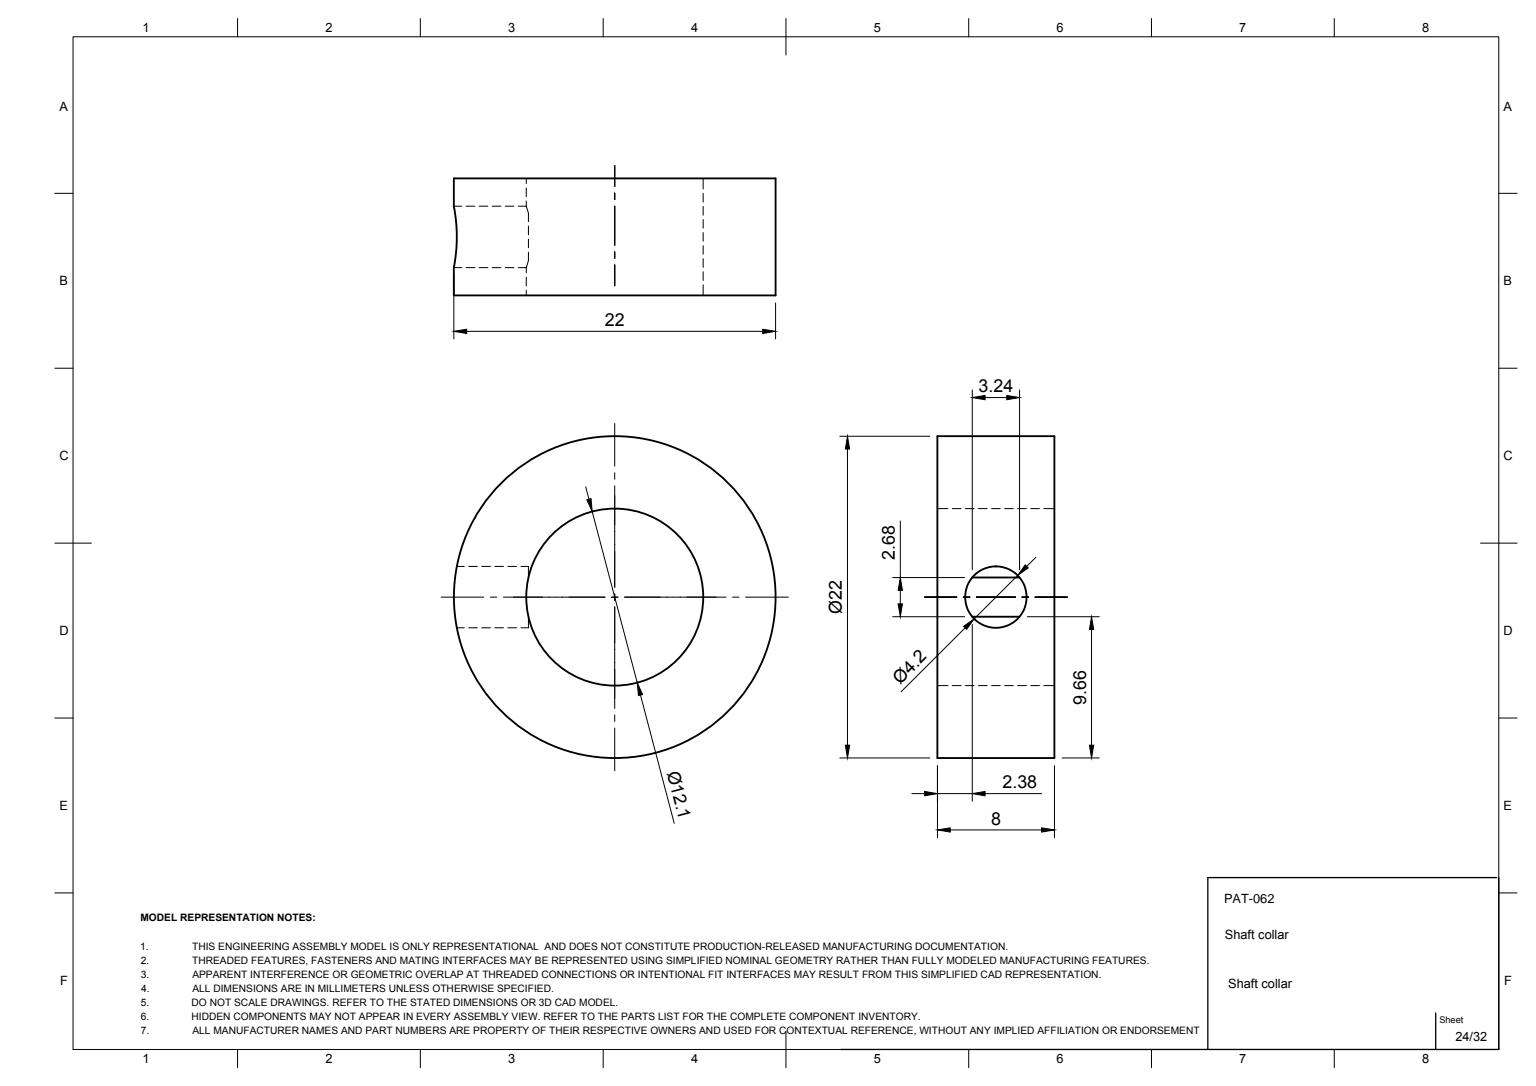
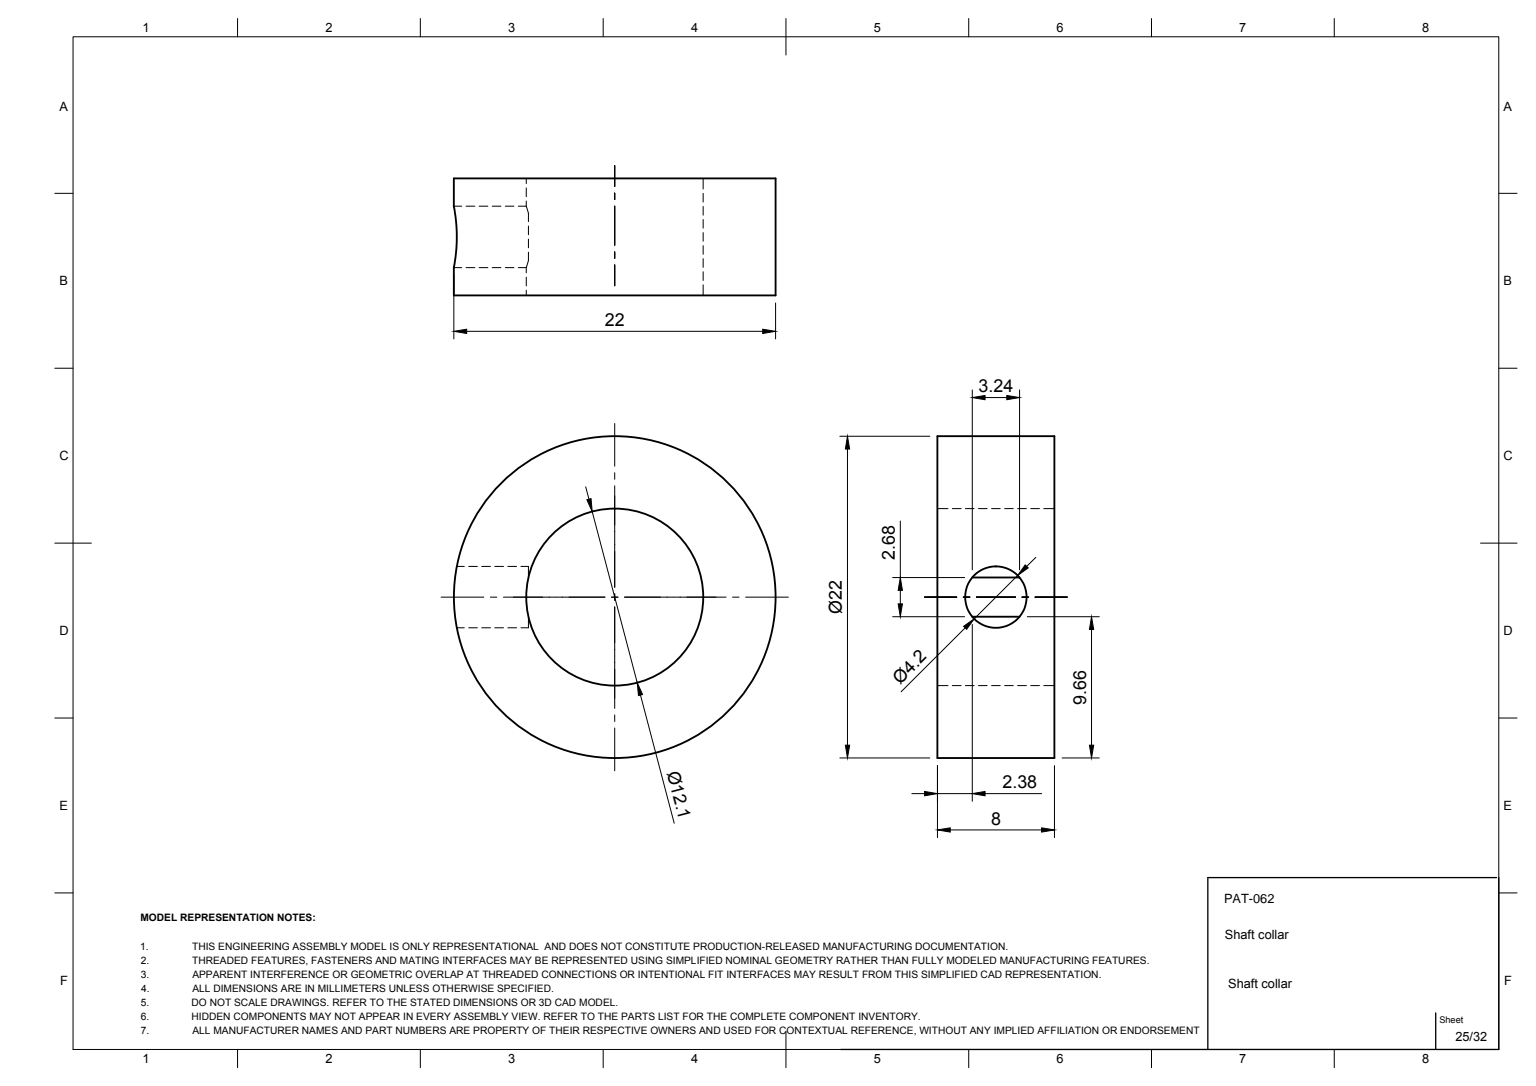
ISO-10303-21;
HEADER;
/* Generated by software containing ST-Developer
 * from STEP Tools, Inc. (www.steptools.com) 
 */

FILE_DESCRIPTION(
/* description */ ('Jaw-coupled motor to shaft test stand'),
/* implementation_level */ '2;1');

FILE_NAME(
/* name */ 'Shaft collar.step',
/* time_stamp */ '2026-10-27T10:46:06-07:00',
/* author */ (''),
/* organization */ (''),
/* preprocessor_version */ 'ST-DEVELOPER v20.2',
/* originating_system */ 'Autodesk Translation Framework v15.17.0.0',
/* authorisation */ '');

FILE_SCHEMA (('AUTOMOTIVE_DESIGN { 1 0 10303 214 3 1 1 }'));
ENDSEC;

DATA;
#10=MECHANICAL_DESIGN_GEOMETRIC_PRESENTATION_REPRESENTATION('',(#363),#19361);
#259=B_SPLINE_CURVE_WITH_KNOTS('',3,(#17076,#17077,#17078,#17079,#17080,
#17081,#17082,#17083,#17084,#17085),.UNSPECIFIED.,.F.,.F.,(4,2,2,2,4),(0.818088904349167,
0.878131747417164,0.957937926194035,1.03774410497091,1.0977869480389),
 .UNSPECIFIED.);
#260=B_SPLINE_CURVE_WITH_KNOTS('',3,(#17091,#17092,#17093,#17094,#17095,
#17096,#17097,#17098,#17099,#17100,#17101,#17102,#17103,#17104,#17105,#17106,
#17107,#17108),.UNSPECIFIED.,.F.,.F.,(4,2,2,2,2,2,2,2,4),(0.,0.0793157643915217,
0.158631528783043,0.237943615933649,0.317255703084255,0.396567790234861,
0.475879877385467,0.555195641776989,0.63451140616851),.UNSPECIFIED.);
#261=B_SPLINE_CURVE_WITH_KNOTS('',3,(#17109,#17110,#17111,#17112,#17113,
#17114,#17115,#17116,#17117,#17118,#17119,#17120,#17121,#17122,#17123,#17124,
#17125,#17126),.UNSPECIFIED.,.F.,.F.,(4,2,2,2,2,2,2,2,4),(0.63451140616851,
0.713827170560032,0.793142934951554,0.87245502210216,0.951767109252766,
1.03107919640337,1.11039128355398,1.1897070479455,1.26902281233702),
 .UNSPECIFIED.);
#262=B_SPLINE_CURVE_WITH_KNOTS('',3,(#17129,#17130,#17131,#17132,#17133,
#17134,#17135,#17136,#17137,#17138),.UNSPECIFIED.,.F.,.F.,(4,2,2,2,4),(0.179463620219811,
0.239506463287807,0.319312642064678,0.399118820841549,0.459161663909546),
 .UNSPECIFIED.);
#298=SHAPE_REPRESENTATION_RELATIONSHIP('SRR','None',#19514,#330);
#330=ADVANCED_BREP_SHAPE_REPRESENTATION('',(#394),#19350);
#363=STYLED_ITEM('',(#19746),#394);
#394=MANIFOLD_SOLID_BREP('Body1',#11009);
#495=FACE_BOUND('',#1973,.T.);
#496=FACE_BOUND('',#1975,.T.);
#497=FACE_BOUND('',#1977,.T.);
#498=FACE_BOUND('',#1979,.T.);
#675=PLANE('',#11808);
#676=PLANE('',#11813);
#677=PLANE('',#11820);
#678=PLANE('',#11821);
#1257=FACE_OUTER_BOUND('',#1969,.T.);
#1258=FACE_OUTER_BOUND('',#1970,.T.);
#1259=FACE_OUTER_BOUND('',#1971,.T.);
#1260=FACE_OUTER_BOUND('',#1972,.T.);
#1261=FACE_OUTER_BOUND('',#1974,.T.);
#1262=FACE_OUTER_BOUND('',#1976,.T.);
#1263=FACE_OUTER_BOUND('',#1978,.T.);
#1969=EDGE_LOOP('',(#8348,#8349));
#1970=EDGE_LOOP('',(#8350,#8351,#8352,#8353,#8354,#8355,#8356,#8357,#8358));
#1971=EDGE_LOOP('',(#8359,#8360,#8361));
#1972=EDGE_LOOP('',(#8362,#8363,#8364,#8365));
#1973=EDGE_LOOP('',(#8366,#8367,#8368,#8369));
#1974=EDGE_LOOP('',(#8370,#8371,#8372,#8373));
#1975=EDGE_LOOP('',(#8374,#8375));
#1976=EDGE_LOOP('',(#8376));
#1977=EDGE_LOOP('',(#8377));
#1978=EDGE_LOOP('',(#8378));
#1979=EDGE_LOOP('',(#8379));
#2698=LINE('',#17072,#3851);
#2699=LINE('',#17089,#3852);
#2700=LINE('',#17140,#3853);
#2701=LINE('',#17145,#3854);
#2702=LINE('',#17151,#3855);
#3851=VECTOR('',#13535,1.);
#3852=VECTOR('',#13542,0.21);
#3853=VECTOR('',#13547,1.);
#3854=VECTOR('',#13552,0.605);
#3855=VECTOR('',#13559,1.1);
#4827=CIRCLE('',#11809,0.21);
#4828=CIRCLE('',#11811,0.21);
#4829=CIRCLE('',#11812,0.21);
#4830=CIRCLE('',#11815,0.605);
#4831=CIRCLE('',#11816,0.605);
#4832=CIRCLE('',#11818,1.1);
#4833=CIRCLE('',#11819,1.1);
#5283=VERTEX_POINT('',#17070);
#5284=VERTEX_POINT('',#17071);
#5285=VERTEX_POINT('',#17075);
#5286=VERTEX_POINT('',#17086);
#5287=VERTEX_POINT('',#17088);
#5288=VERTEX_POINT('',#17090);
#5289=VERTEX_POINT('',#17127);
#5290=VERTEX_POINT('',#17142);
#5291=VERTEX_POINT('',#17144);
#5292=VERTEX_POINT('',#17148);
#5293=VERTEX_POINT('',#17150);
#6385=EDGE_CURVE('',#5283,#5284,#2698,.T.);
#6386=EDGE_CURVE('',#5283,#5284,#4827,.T.);
#6387=EDGE_CURVE('',#5285,#5283,#259,.T.);
#6388=EDGE_CURVE('',#5286,#5285,#4828,.T.);
#6389=EDGE_CURVE('',#5286,#5287,#2699,.T.);
#6390=EDGE_CURVE('',#5288,#5287,#260,.T.);
#6391=EDGE_CURVE('',#5287,#5288,#261,.T.);
#6392=EDGE_CURVE('',#5289,#5286,#4829,.T.);
#6393=EDGE_CURVE('',#5284,#5289,#262,.T.);
#6394=EDGE_CURVE('',#5289,#5285,#2700,.T.);
#6395=EDGE_CURVE('',#5290,#5290,#4830,.T.);
#6396=EDGE_CURVE('',#5290,#5291,#2701,.T.);
#6397=EDGE_CURVE('',#5291,#5291,#4831,.T.);
#6398=EDGE_CURVE('',#5292,#5292,#4832,.T.);
#6399=EDGE_CURVE('',#5292,#5293,#2702,.T.);
#6400=EDGE_CURVE('',#5293,#5293,#4833,.T.);
#8348=ORIENTED_EDGE('',*,*,#6385,.F.);
#8349=ORIENTED_EDGE('',*,*,#6386,.T.);
#8350=ORIENTED_EDGE('',*,*,#6387,.F.);
#8351=ORIENTED_EDGE('',*,*,#6388,.F.);
#8352=ORIENTED_EDGE('',*,*,#6389,.T.);
#8353=ORIENTED_EDGE('',*,*,#6390,.F.);
#8354=ORIENTED_EDGE('',*,*,#6391,.F.);
#8355=ORIENTED_EDGE('',*,*,#6389,.F.);
#8356=ORIENTED_EDGE('',*,*,#6392,.F.);
#8357=ORIENTED_EDGE('',*,*,#6393,.F.);
#8358=ORIENTED_EDGE('',*,*,#6386,.F.);
#8359=ORIENTED_EDGE('',*,*,#6394,.F.);
#8360=ORIENTED_EDGE('',*,*,#6392,.T.);
#8361=ORIENTED_EDGE('',*,*,#6388,.T.);
#8362=ORIENTED_EDGE('',*,*,#6395,.F.);
#8363=ORIENTED_EDGE('',*,*,#6396,.T.);
#8364=ORIENTED_EDGE('',*,*,#6397,.T.);
#8365=ORIENTED_EDGE('',*,*,#6396,.F.);
#8366=ORIENTED_EDGE('',*,*,#6393,.T.);
#8367=ORIENTED_EDGE('',*,*,#6394,.T.);
#8368=ORIENTED_EDGE('',*,*,#6387,.T.);
#8369=ORIENTED_EDGE('',*,*,#6385,.T.);
#8370=ORIENTED_EDGE('',*,*,#6398,.F.);
#8371=ORIENTED_EDGE('',*,*,#6399,.T.);
#8372=ORIENTED_EDGE('',*,*,#6400,.T.);
#8373=ORIENTED_EDGE('',*,*,#6399,.F.);
#8374=ORIENTED_EDGE('',*,*,#6390,.T.);
#8375=ORIENTED_EDGE('',*,*,#6391,.T.);
#8376=ORIENTED_EDGE('',*,*,#6398,.T.);
#8377=ORIENTED_EDGE('',*,*,#6395,.T.);
#8378=ORIENTED_EDGE('',*,*,#6400,.F.);
#8379=ORIENTED_EDGE('',*,*,#6397,.F.);
#10338=CYLINDRICAL_SURFACE('',#11810,0.21);
#10339=CYLINDRICAL_SURFACE('',#11814,0.605);
#10340=CYLINDRICAL_SURFACE('',#11817,1.1);
#10599=ADVANCED_FACE('',(#1257),#675,.T.);
#10600=ADVANCED_FACE('',(#1258),#10338,.F.);
#10601=ADVANCED_FACE('',(#1259),#676,.T.);
#10602=ADVANCED_FACE('',(#1260,#495),#10339,.F.);
#10603=ADVANCED_FACE('',(#1261,#496),#10340,.T.);
#10604=ADVANCED_FACE('',(#1262,#497),#677,.T.);
#10605=ADVANCED_FACE('',(#1263,#498),#678,.F.);
#11009=CLOSED_SHELL('',(#10599,#10600,#10601,#10602,#10603,#10604,#10605));
#11807=AXIS2_PLACEMENT_3D('',#17068,#13531,#13532);
#11808=AXIS2_PLACEMENT_3D('',#17069,#13533,#13534);
#11809=AXIS2_PLACEMENT_3D('',#17073,#13536,#13537);
#11810=AXIS2_PLACEMENT_3D('',#17074,#13538,#13539);
#11811=AXIS2_PLACEMENT_3D('',#17087,#13540,#13541);
#11812=AXIS2_PLACEMENT_3D('',#17128,#13543,#13544);
#11813=AXIS2_PLACEMENT_3D('',#17139,#13545,#13546);
#11814=AXIS2_PLACEMENT_3D('',#17141,#13548,#13549);
#11815=AXIS2_PLACEMENT_3D('',#17143,#13550,#13551);
#11816=AXIS2_PLACEMENT_3D('',#17146,#13553,#13554);
#11817=AXIS2_PLACEMENT_3D('',#17147,#13555,#13556);
#11818=AXIS2_PLACEMENT_3D('',#17149,#13557,#13558);
#11819=AXIS2_PLACEMENT_3D('',#17152,#13560,#13561);
#11820=AXIS2_PLACEMENT_3D('',#17153,#13562,#13563);
#11821=AXIS2_PLACEMENT_3D('',#17154,#13564,#13565);
#13531=DIRECTION('axis',(0.,0.,1.));
#13532=DIRECTION('refdir',(1.,0.,0.));
#13533=DIRECTION('center_axis',(0.,0.,1.));
#13534=DIRECTION('ref_axis',(1.,0.,0.));
#13535=DIRECTION('',(0.,1.,0.));
#13536=DIRECTION('center_axis',(0.,0.,1.));
#13537=DIRECTION('ref_axis',(1.,0.,0.));
#13538=DIRECTION('center_axis',(0.,0.,1.));
#13539=DIRECTION('ref_axis',(1.,0.,0.));
#13540=DIRECTION('center_axis',(0.,0.,1.));
#13541=DIRECTION('ref_axis',(1.,0.,0.));
#13542=DIRECTION('',(0.,0.,1.));
#13543=DIRECTION('center_axis',(0.,0.,1.));
#13544=DIRECTION('ref_axis',(1.,0.,0.));
#13545=DIRECTION('center_axis',(0.,0.,1.));
#13546=DIRECTION('ref_axis',(1.,0.,0.));
#13547=DIRECTION('',(0.,-1.,0.));
#13548=DIRECTION('center_axis',(0.,1.,0.));
#13549=DIRECTION('ref_axis',(1.,0.,0.));
#13550=DIRECTION('center_axis',(0.,-1.,0.));
#13551=DIRECTION('ref_axis',(1.,0.,0.));
#13552=DIRECTION('',(0.,-1.,0.));
#13553=DIRECTION('center_axis',(0.,-1.,0.));
#13554=DIRECTION('ref_axis',(1.,0.,0.));
#13555=DIRECTION('center_axis',(0.,1.,0.));
#13556=DIRECTION('ref_axis',(1.,0.,0.));
#13557=DIRECTION('center_axis',(0.,1.,0.));
#13558=DIRECTION('ref_axis',(1.,0.,0.));
#13559=DIRECTION('',(0.,-1.,0.));
#13560=DIRECTION('center_axis',(0.,1.,0.));
#13561=DIRECTION('ref_axis',(1.,0.,0.));
#13562=DIRECTION('center_axis',(0.,1.,0.));
#13563=DIRECTION('ref_axis',(1.,0.,0.));
#13564=DIRECTION('center_axis',(0.,1.,0.));
#13565=DIRECTION('ref_axis',(1.,0.,0.));
#17068=CARTESIAN_POINT('',(0.,0.,0.));
#17069=CARTESIAN_POINT('Origin',(0.,0.75,4.81));
#17070=CARTESIAN_POINT('',(0.133884278389959,0.588213103126366,4.81));
#17071=CARTESIAN_POINT('',(0.133884278389959,0.911786896873634,4.81));
#17072=CARTESIAN_POINT('',(0.133884278389959,0.35,4.81));
#17073=CARTESIAN_POINT('Origin',(0.,0.75,4.81));
#17074=CARTESIAN_POINT('Origin',(0.,0.75,4.81));
#17075=CARTESIAN_POINT('',(-0.133884278389959,0.588213103126366,4.81));
#17076=CARTESIAN_POINT('Ctrl Pts',(-0.133884278389959,0.588213103126366,
4.81));
#17077=CARTESIAN_POINT('Ctrl Pts',(-0.118254395260805,0.575278831782373,
4.81354677224418));
#17078=CARTESIAN_POINT('Ctrl Pts',(-0.1001097876823,0.564200683412563,4.81698224789957));
#17079=CARTESIAN_POINT('Ctrl Pts',(-0.0548298721325192,0.545361438945571,
4.8230741628997));
#17080=CARTESIAN_POINT('Ctrl Pts',(-0.0266020595922903,0.54,4.825));
#17081=CARTESIAN_POINT('Ctrl Pts',(0.0266020595922903,0.54,4.825));
#17082=CARTESIAN_POINT('Ctrl Pts',(0.0548298721325192,0.545361438945571,
4.8230741628997));
#17083=CARTESIAN_POINT('Ctrl Pts',(0.1001097876823,0.564200683412563,4.81698224789957));
#17084=CARTESIAN_POINT('Ctrl Pts',(0.118254395260805,0.575278831782372,
4.81354677224418));
#17085=CARTESIAN_POINT('Ctrl Pts',(0.133884278389959,0.588213103126366,
4.81));
#17086=CARTESIAN_POINT('',(-0.21,0.75,4.81));
#17087=CARTESIAN_POINT('Origin',(0.,0.75,4.81));
#17088=CARTESIAN_POINT('',(-0.21,0.75,5.29976849370594));
#17089=CARTESIAN_POINT('',(-0.21,0.75,4.81));
#17090=CARTESIAN_POINT('',(0.21,0.75,5.29976849370594));
#17091=CARTESIAN_POINT('Ctrl Pts',(0.21,0.75,5.29976849370594));
#17092=CARTESIAN_POINT('Ctrl Pts',(0.21,0.723561411869493,5.29976849370594));
#17093=CARTESIAN_POINT('Ctrl Pts',(0.204702922670976,0.695406218745069,
5.30084015664674));
#17094=CARTESIAN_POINT('Ctrl Pts',(0.183251796806354,0.643686554458656,
5.30468313707126));
#17095=CARTESIAN_POINT('Ctrl Pts',(0.167101177357214,0.620116329258865,
5.30739593054622));
#17096=CARTESIAN_POINT('Ctrl Pts',(0.129884533480965,0.582899685382615,
5.31246633289124));
#17097=CARTESIAN_POINT('Ctrl Pts',(0.106313940757289,0.566748389836589,
5.31515738895358));
#17098=CARTESIAN_POINT('Ctrl Pts',(0.0545930033295205,0.545296773430262,
5.31895039220591));
#17099=CARTESIAN_POINT('Ctrl Pts',(0.0264373623835353,0.54,5.32));
#17100=CARTESIAN_POINT('Ctrl Pts',(-0.0264373623835353,0.54,5.32));
#17101=CARTESIAN_POINT('Ctrl Pts',(-0.0545930033295205,0.545296773430262,
5.31895039220591));
#17102=CARTESIAN_POINT('Ctrl Pts',(-0.106313940757289,0.566748389836589,
5.31515738895358));
#17103=CARTESIAN_POINT('Ctrl Pts',(-0.129884533480965,0.582899685382615,
5.31246633289124));
#17104=CARTESIAN_POINT('Ctrl Pts',(-0.167101177357214,0.620116329258865,
5.30739593054622));
#17105=CARTESIAN_POINT('Ctrl Pts',(-0.183251796806354,0.643686554458656,
5.30468313707126));
#17106=CARTESIAN_POINT('Ctrl Pts',(-0.204702922670976,0.695406218745069,
5.30084015664674));
#17107=CARTESIAN_POINT('Ctrl Pts',(-0.21,0.723561411869493,5.29976849370594));
#17108=CARTESIAN_POINT('Ctrl Pts',(-0.21,0.75,5.29976849370594));
#17109=CARTESIAN_POINT('Ctrl Pts',(-0.21,0.75,5.29976849370594));
#17110=CARTESIAN_POINT('Ctrl Pts',(-0.21,0.776438588130507,5.29976849370594));
#17111=CARTESIAN_POINT('Ctrl Pts',(-0.204702922670976,0.804593781254931,
5.30084015664674));
#17112=CARTESIAN_POINT('Ctrl Pts',(-0.183251796806354,0.856313445541343,
5.30468313707126));
#17113=CARTESIAN_POINT('Ctrl Pts',(-0.167101177357215,0.879883670741135,
5.30739593054622));
#17114=CARTESIAN_POINT('Ctrl Pts',(-0.129884533480965,0.917100314617385,
5.31246633289124));
#17115=CARTESIAN_POINT('Ctrl Pts',(-0.106313940757289,0.933251610163411,
5.31515738895358));
#17116=CARTESIAN_POINT('Ctrl Pts',(-0.0545930033295205,0.954703226569738,
5.31895039220591));
#17117=CARTESIAN_POINT('Ctrl Pts',(-0.0264373623835353,0.96,5.32));
#17118=CARTESIAN_POINT('Ctrl Pts',(0.0264373623835353,0.96,5.32));
#17119=CARTESIAN_POINT('Ctrl Pts',(0.0545930033295204,0.954703226569738,
5.31895039220591));
#17120=CARTESIAN_POINT('Ctrl Pts',(0.106313940757288,0.933251610163411,
5.31515738895358));
#17121=CARTESIAN_POINT('Ctrl Pts',(0.129884533480965,0.917100314617385,
5.31246633289124));
#17122=CARTESIAN_POINT('Ctrl Pts',(0.167101177357214,0.879883670741136,
5.30739593054622));
#17123=CARTESIAN_POINT('Ctrl Pts',(0.183251796806354,0.856313445541344,
5.30468313707126));
#17124=CARTESIAN_POINT('Ctrl Pts',(0.204702922670976,0.804593781254931,
5.30084015664674));
#17125=CARTESIAN_POINT('Ctrl Pts',(0.21,0.776438588130507,5.29976849370594));
#17126=CARTESIAN_POINT('Ctrl Pts',(0.21,0.75,5.29976849370594));
#17127=CARTESIAN_POINT('',(-0.133884278389959,0.911786896873634,4.81));
#17128=CARTESIAN_POINT('Origin',(0.,0.75,4.81));
#17129=CARTESIAN_POINT('Ctrl Pts',(0.133884278389959,0.911786896873634,
4.81));
#17130=CARTESIAN_POINT('Ctrl Pts',(0.118254395260805,0.924721168217627,
4.81354677224418));
#17131=CARTESIAN_POINT('Ctrl Pts',(0.1001097876823,0.935799316587437,4.81698224789957));
#17132=CARTESIAN_POINT('Ctrl Pts',(0.0548298721325192,0.954638561054429,
4.8230741628997));
#17133=CARTESIAN_POINT('Ctrl Pts',(0.0266020595922903,0.96,4.825));
#17134=CARTESIAN_POINT('Ctrl Pts',(-0.0266020595922903,0.96,4.825));
#17135=CARTESIAN_POINT('Ctrl Pts',(-0.0548298721325192,0.954638561054429,
4.8230741628997));
#17136=CARTESIAN_POINT('Ctrl Pts',(-0.1001097876823,0.935799316587437,4.81698224789957));
#17137=CARTESIAN_POINT('Ctrl Pts',(-0.118254395260804,0.924721168217628,
4.81354677224418));
#17138=CARTESIAN_POINT('Ctrl Pts',(-0.133884278389959,0.911786896873634,
4.81));
#17139=CARTESIAN_POINT('Origin',(0.,0.75,4.81));
#17140=CARTESIAN_POINT('',(-0.133884278389959,0.35,4.81));
#17141=CARTESIAN_POINT('Origin',(0.,0.35,4.22));
#17142=CARTESIAN_POINT('',(-0.605,1.15,4.22));
#17143=CARTESIAN_POINT('Origin',(0.,1.15,4.22));
#17144=CARTESIAN_POINT('',(-0.605,0.35,4.22));
#17145=CARTESIAN_POINT('',(-0.605,0.35,4.22));
#17146=CARTESIAN_POINT('Origin',(0.,0.35,4.22));
#17147=CARTESIAN_POINT('Origin',(0.,0.35,4.22));
#17148=CARTESIAN_POINT('',(-1.1,1.15,4.22));
#17149=CARTESIAN_POINT('Origin',(0.,1.15,4.22));
#17150=CARTESIAN_POINT('',(-1.1,0.35,4.22));
#17151=CARTESIAN_POINT('',(-1.1,0.35,4.22));
#17152=CARTESIAN_POINT('Origin',(0.,0.35,4.22));
#17153=CARTESIAN_POINT('Origin',(0.,1.15,4.22));
#17154=CARTESIAN_POINT('Origin',(0.,0.35,4.22));
#19312=UNCERTAINTY_MEASURE_WITH_UNIT(LENGTH_MEASURE(0.001),#19362,
'DISTANCE_ACCURACY_VALUE',
'Maximum model space distance between geometric entities at asserted c
onnectivities');
#19323=UNCERTAINTY_MEASURE_WITH_UNIT(LENGTH_MEASURE(0.001),#19362,
'DISTANCE_ACCURACY_VALUE',
'Maximum model space distance between geometric entities at asserted c
onnectivities');
#19350=(
GEOMETRIC_REPRESENTATION_CONTEXT(3)
GLOBAL_UNCERTAINTY_ASSIGNED_CONTEXT((#19312))
GLOBAL_UNIT_ASSIGNED_CONTEXT((#19362,#19364,#19365))
REPRESENTATION_CONTEXT('','3D')
);
#19361=(
GEOMETRIC_REPRESENTATION_CONTEXT(3)
GLOBAL_UNCERTAINTY_ASSIGNED_CONTEXT((#19323))
GLOBAL_UNIT_ASSIGNED_CONTEXT((#19362,#19364,#19365))
REPRESENTATION_CONTEXT('','3D')
);
#19362=(
LENGTH_UNIT()
NAMED_UNIT(*)
SI_UNIT(.CENTI.,.METRE.)
);
#19364=(
NAMED_UNIT(*)
PLANE_ANGLE_UNIT()
SI_UNIT($,.RADIAN.)
);
#19365=(
NAMED_UNIT(*)
SI_UNIT($,.STERADIAN.)
SOLID_ANGLE_UNIT()
);
#19392=SHAPE_DEFINITION_REPRESENTATION(#19456,#19514);
#19456=PRODUCT_DEFINITION_SHAPE('',$,#19552);
#19514=SHAPE_REPRESENTATION('',(#11807),#19350);
#19525=PRODUCT_DEFINITION_CONTEXT('part definition',#19638,'design');
#19552=PRODUCT_DEFINITION('Shaft collar','Shaft collar',#19589,#19525);
#19589=PRODUCT_DEFINITION_FORMATION('',$,#19666);
#19638=APPLICATION_CONTEXT(
'Core Data for Automotive Mechanical Design Process');
#19639=PRODUCT_CONTEXT('part definition',#19638,'mechanical');
#19666=PRODUCT('Shaft collar','Shaft collar','Shaft collar',(#19639));
#19740=COLOUR_RGB('Grey',0.48,0.52,0.57);
#19741=FILL_AREA_STYLE_COLOUR('',#19740);
#19742=FILL_AREA_STYLE('',(#19741));
#19743=SURFACE_STYLE_FILL_AREA(#19742);
#19744=SURFACE_SIDE_STYLE('',(#19743));
#19745=SURFACE_STYLE_USAGE(.BOTH.,#19744);
#19746=PRESENTATION_STYLE_ASSIGNMENT((#19745));
ENDSEC;
END-ISO-10303-21;
